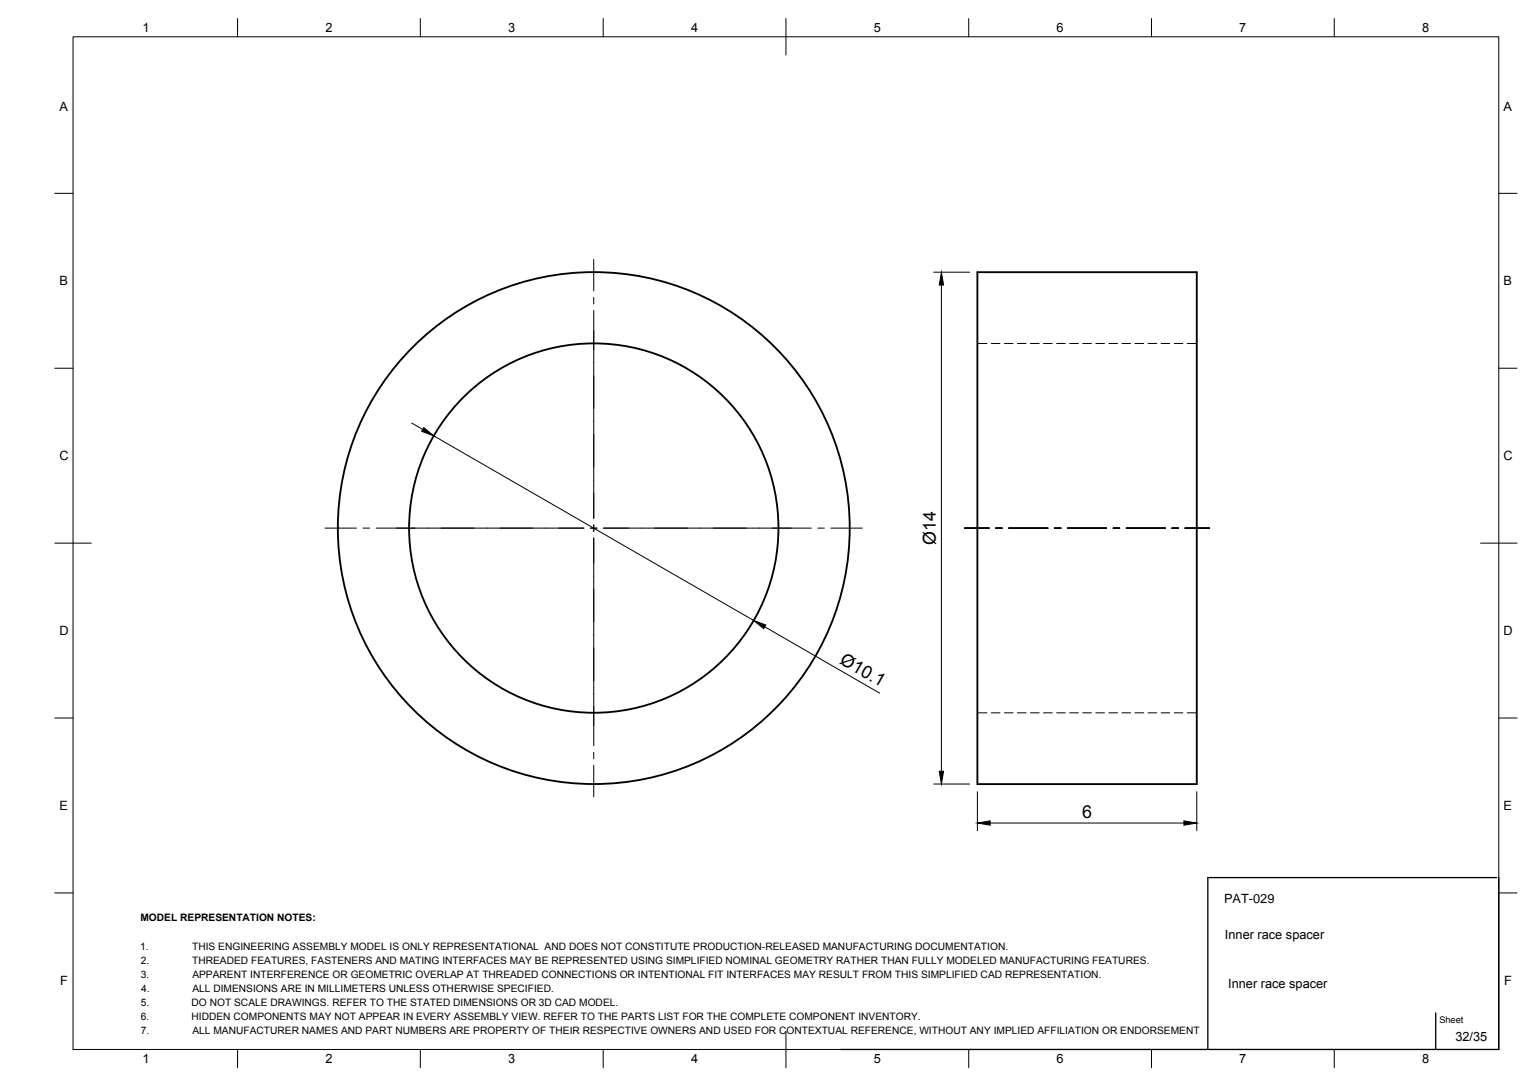
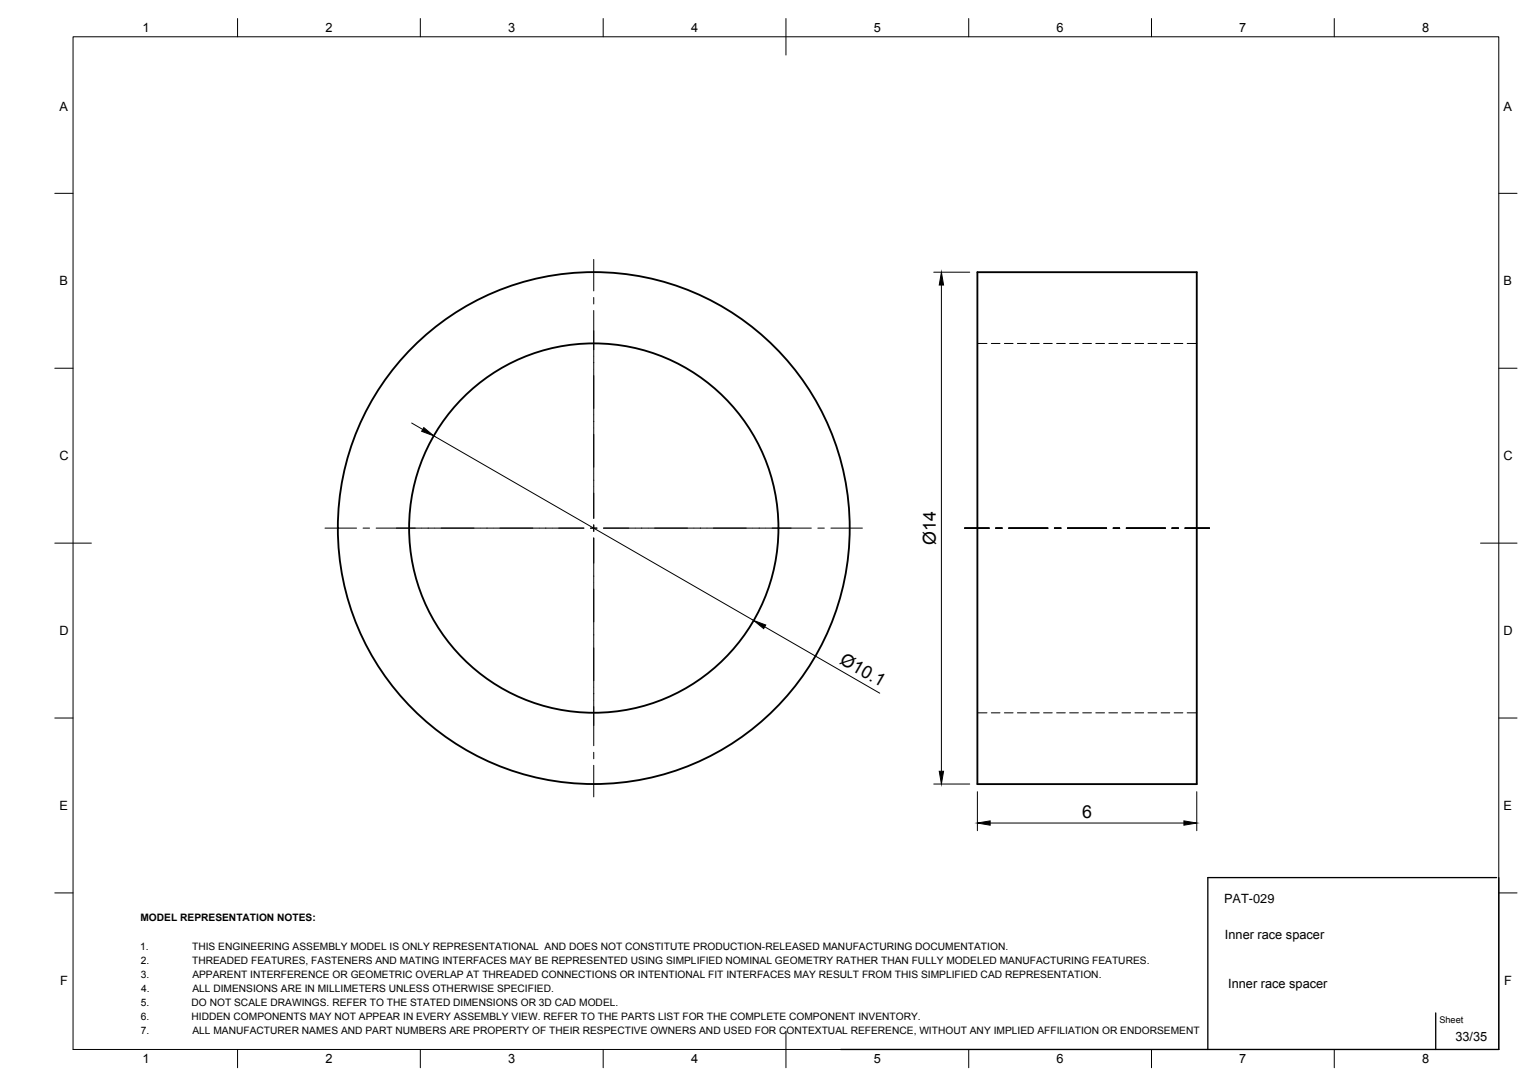
ISO-10303-21;
HEADER;
/* Generated by software containing ST-Developer
 * from STEP Tools, Inc. (www.steptools.com) 
 */

FILE_DESCRIPTION(
/* description */ ('Door-style hinge test fixture with detent'),
/* implementation_level */ '2;1');

FILE_NAME(
/* name */ 'Inner race spacer.step',
/* time_stamp */ '2026-10-28T03:24:57-07:00',
/* author */ (''),
/* organization */ (''),
/* preprocessor_version */ 'ST-DEVELOPER v20.2',
/* originating_system */ 'Autodesk Translation Framework v15.17.0.0',
/* authorisation */ '');

FILE_SCHEMA (('AUTOMOTIVE_DESIGN { 1 0 10303 214 3 1 1 }'));
ENDSEC;

DATA;
#10=MECHANICAL_DESIGN_GEOMETRIC_PRESENTATION_REPRESENTATION('',(#357),#9813);
#286=SHAPE_REPRESENTATION_RELATIONSHIP('SRR','None',#9965,#317);
#317=ADVANCED_BREP_SHAPE_REPRESENTATION('',(#395),#9808);
#357=STYLED_ITEM('',(#10183),#395);
#395=MANIFOLD_SOLID_BREP('Body1',#4790);
#491=FACE_BOUND('',#1295,.T.);
#492=FACE_BOUND('',#1297,.T.);
#644=PLANE('',#5687);
#645=PLANE('',#5688);
#915=FACE_OUTER_BOUND('',#1292,.T.);
#916=FACE_OUTER_BOUND('',#1293,.T.);
#917=FACE_OUTER_BOUND('',#1294,.T.);
#918=FACE_OUTER_BOUND('',#1296,.T.);
#1292=EDGE_LOOP('',(#4269,#4270,#4271,#4272));
#1293=EDGE_LOOP('',(#4273,#4274,#4275,#4276));
#1294=EDGE_LOOP('',(#4277));
#1295=EDGE_LOOP('',(#4278));
#1296=EDGE_LOOP('',(#4279));
#1297=EDGE_LOOP('',(#4280));
#1622=LINE('',#9608,#1942);
#1623=LINE('',#9614,#1943);
#1942=VECTOR('',#7129,0.505);
#1943=VECTOR('',#7136,0.7);
#2197=CIRCLE('',#5682,0.505);
#2198=CIRCLE('',#5683,0.505);
#2199=CIRCLE('',#5685,0.7);
#2200=CIRCLE('',#5686,0.7);
#2584=VERTEX_POINT('',#9605);
#2585=VERTEX_POINT('',#9607);
#2586=VERTEX_POINT('',#9611);
#2587=VERTEX_POINT('',#9613);
#3151=EDGE_CURVE('',#2584,#2584,#2197,.T.);
#3152=EDGE_CURVE('',#2584,#2585,#1622,.T.);
#3153=EDGE_CURVE('',#2585,#2585,#2198,.T.);
#3154=EDGE_CURVE('',#2586,#2586,#2199,.T.);
#3155=EDGE_CURVE('',#2586,#2587,#1623,.T.);
#3156=EDGE_CURVE('',#2587,#2587,#2200,.T.);
#4269=ORIENTED_EDGE('',*,*,#3151,.F.);
#4270=ORIENTED_EDGE('',*,*,#3152,.T.);
#4271=ORIENTED_EDGE('',*,*,#3153,.T.);
#4272=ORIENTED_EDGE('',*,*,#3152,.F.);
#4273=ORIENTED_EDGE('',*,*,#3154,.F.);
#4274=ORIENTED_EDGE('',*,*,#3155,.T.);
#4275=ORIENTED_EDGE('',*,*,#3156,.T.);
#4276=ORIENTED_EDGE('',*,*,#3155,.F.);
#4277=ORIENTED_EDGE('',*,*,#3154,.T.);
#4278=ORIENTED_EDGE('',*,*,#3151,.T.);
#4279=ORIENTED_EDGE('',*,*,#3156,.F.);
#4280=ORIENTED_EDGE('',*,*,#3153,.F.);
#4458=CYLINDRICAL_SURFACE('',#5681,0.505);
#4459=CYLINDRICAL_SURFACE('',#5684,0.7);
#4720=ADVANCED_FACE('',(#915),#4458,.F.);
#4721=ADVANCED_FACE('',(#916),#4459,.T.);
#4722=ADVANCED_FACE('',(#917,#491),#644,.T.);
#4723=ADVANCED_FACE('',(#918,#492),#645,.F.);
#4790=CLOSED_SHELL('',(#4720,#4721,#4722,#4723));
#5680=AXIS2_PLACEMENT_3D('',#9603,#7123,#7124);
#5681=AXIS2_PLACEMENT_3D('',#9604,#7125,#7126);
#5682=AXIS2_PLACEMENT_3D('',#9606,#7127,#7128);
#5683=AXIS2_PLACEMENT_3D('',#9609,#7130,#7131);
#5684=AXIS2_PLACEMENT_3D('',#9610,#7132,#7133);
#5685=AXIS2_PLACEMENT_3D('',#9612,#7134,#7135);
#5686=AXIS2_PLACEMENT_3D('',#9615,#7137,#7138);
#5687=AXIS2_PLACEMENT_3D('',#9616,#7139,#7140);
#5688=AXIS2_PLACEMENT_3D('',#9617,#7141,#7142);
#7123=DIRECTION('axis',(0.,0.,1.));
#7124=DIRECTION('refdir',(1.,0.,0.));
#7125=DIRECTION('center_axis',(0.,0.,1.));
#7126=DIRECTION('ref_axis',(1.,0.,0.));
#7127=DIRECTION('center_axis',(0.,0.,-1.));
#7128=DIRECTION('ref_axis',(1.,0.,0.));
#7129=DIRECTION('',(0.,0.,-1.));
#7130=DIRECTION('center_axis',(0.,0.,-1.));
#7131=DIRECTION('ref_axis',(1.,0.,0.));
#7132=DIRECTION('center_axis',(0.,0.,1.));
#7133=DIRECTION('ref_axis',(1.,0.,0.));
#7134=DIRECTION('center_axis',(0.,0.,1.));
#7135=DIRECTION('ref_axis',(1.,0.,0.));
#7136=DIRECTION('',(0.,0.,-1.));
#7137=DIRECTION('center_axis',(0.,0.,1.));
#7138=DIRECTION('ref_axis',(1.,0.,0.));
#7139=DIRECTION('center_axis',(0.,0.,1.));
#7140=DIRECTION('ref_axis',(1.,0.,0.));
#7141=DIRECTION('center_axis',(0.,0.,1.));
#7142=DIRECTION('ref_axis',(1.,0.,0.));
#9603=CARTESIAN_POINT('',(0.,0.,0.));
#9604=CARTESIAN_POINT('Origin',(0.,0.,3.4));
#9605=CARTESIAN_POINT('',(-0.505,-6.18446633569413E-17,4.));
#9606=CARTESIAN_POINT('Origin',(0.,0.,4.));
#9607=CARTESIAN_POINT('',(-0.505,-6.18446633569413E-17,3.4));
#9608=CARTESIAN_POINT('',(-0.505,-6.18446633569413E-17,3.4));
#9609=CARTESIAN_POINT('Origin',(0.,0.,3.4));
#9610=CARTESIAN_POINT('Origin',(0.,0.,3.4));
#9611=CARTESIAN_POINT('',(-0.7,-8.57252759403147E-17,4.));
#9612=CARTESIAN_POINT('Origin',(0.,0.,4.));
#9613=CARTESIAN_POINT('',(-0.7,-8.57252759403147E-17,3.4));
#9614=CARTESIAN_POINT('',(-0.7,-8.57252759403147E-17,3.4));
#9615=CARTESIAN_POINT('Origin',(0.,0.,3.4));
#9616=CARTESIAN_POINT('Origin',(0.,0.,4.));
#9617=CARTESIAN_POINT('Origin',(0.,0.,3.4));
#9772=UNCERTAINTY_MEASURE_WITH_UNIT(LENGTH_MEASURE(0.001),#9814,
'DISTANCE_ACCURACY_VALUE',
'Maximum model space distance between geometric entities at asserted c
onnectivities');
#9777=UNCERTAINTY_MEASURE_WITH_UNIT(LENGTH_MEASURE(0.001),#9814,
'DISTANCE_ACCURACY_VALUE',
'Maximum model space distance between geometric entities at asserted c
onnectivities');
#9808=(
GEOMETRIC_REPRESENTATION_CONTEXT(3)
GLOBAL_UNCERTAINTY_ASSIGNED_CONTEXT((#9772))
GLOBAL_UNIT_ASSIGNED_CONTEXT((#9814,#9816,#9817))
REPRESENTATION_CONTEXT('','3D')
);
#9813=(
GEOMETRIC_REPRESENTATION_CONTEXT(3)
GLOBAL_UNCERTAINTY_ASSIGNED_CONTEXT((#9777))
GLOBAL_UNIT_ASSIGNED_CONTEXT((#9814,#9816,#9817))
REPRESENTATION_CONTEXT('','3D')
);
#9814=(
LENGTH_UNIT()
NAMED_UNIT(*)
SI_UNIT(.CENTI.,.METRE.)
);
#9816=(
NAMED_UNIT(*)
PLANE_ANGLE_UNIT()
SI_UNIT($,.RADIAN.)
);
#9817=(
NAMED_UNIT(*)
SI_UNIT($,.STERADIAN.)
SOLID_ANGLE_UNIT()
);
#9848=SHAPE_DEFINITION_REPRESENTATION(#9921,#9965);
#9921=PRODUCT_DEFINITION_SHAPE('',$,#10001);
#9965=SHAPE_REPRESENTATION('',(#5680),#9808);
#9970=PRODUCT_DEFINITION_CONTEXT('part definition',#10077,'design');
#10001=PRODUCT_DEFINITION('Inner race spacer','Inner race spacer',#10036,
#9970);
#10036=PRODUCT_DEFINITION_FORMATION('',$,#10109);
#10077=APPLICATION_CONTEXT(
'Core Data for Automotive Mechanical Design Process');
#10078=PRODUCT_CONTEXT('part definition',#10077,'mechanical');
#10109=PRODUCT('Inner race spacer','Inner race spacer',
'Inner race spacer',(#10078));
#10177=COLOUR_RGB('Grey',0.48,0.52,0.57);
#10178=FILL_AREA_STYLE_COLOUR('',#10177);
#10179=FILL_AREA_STYLE('',(#10178));
#10180=SURFACE_STYLE_FILL_AREA(#10179);
#10181=SURFACE_SIDE_STYLE('',(#10180));
#10182=SURFACE_STYLE_USAGE(.BOTH.,#10181);
#10183=PRESENTATION_STYLE_ASSIGNMENT((#10182));
ENDSEC;
END-ISO-10303-21;
